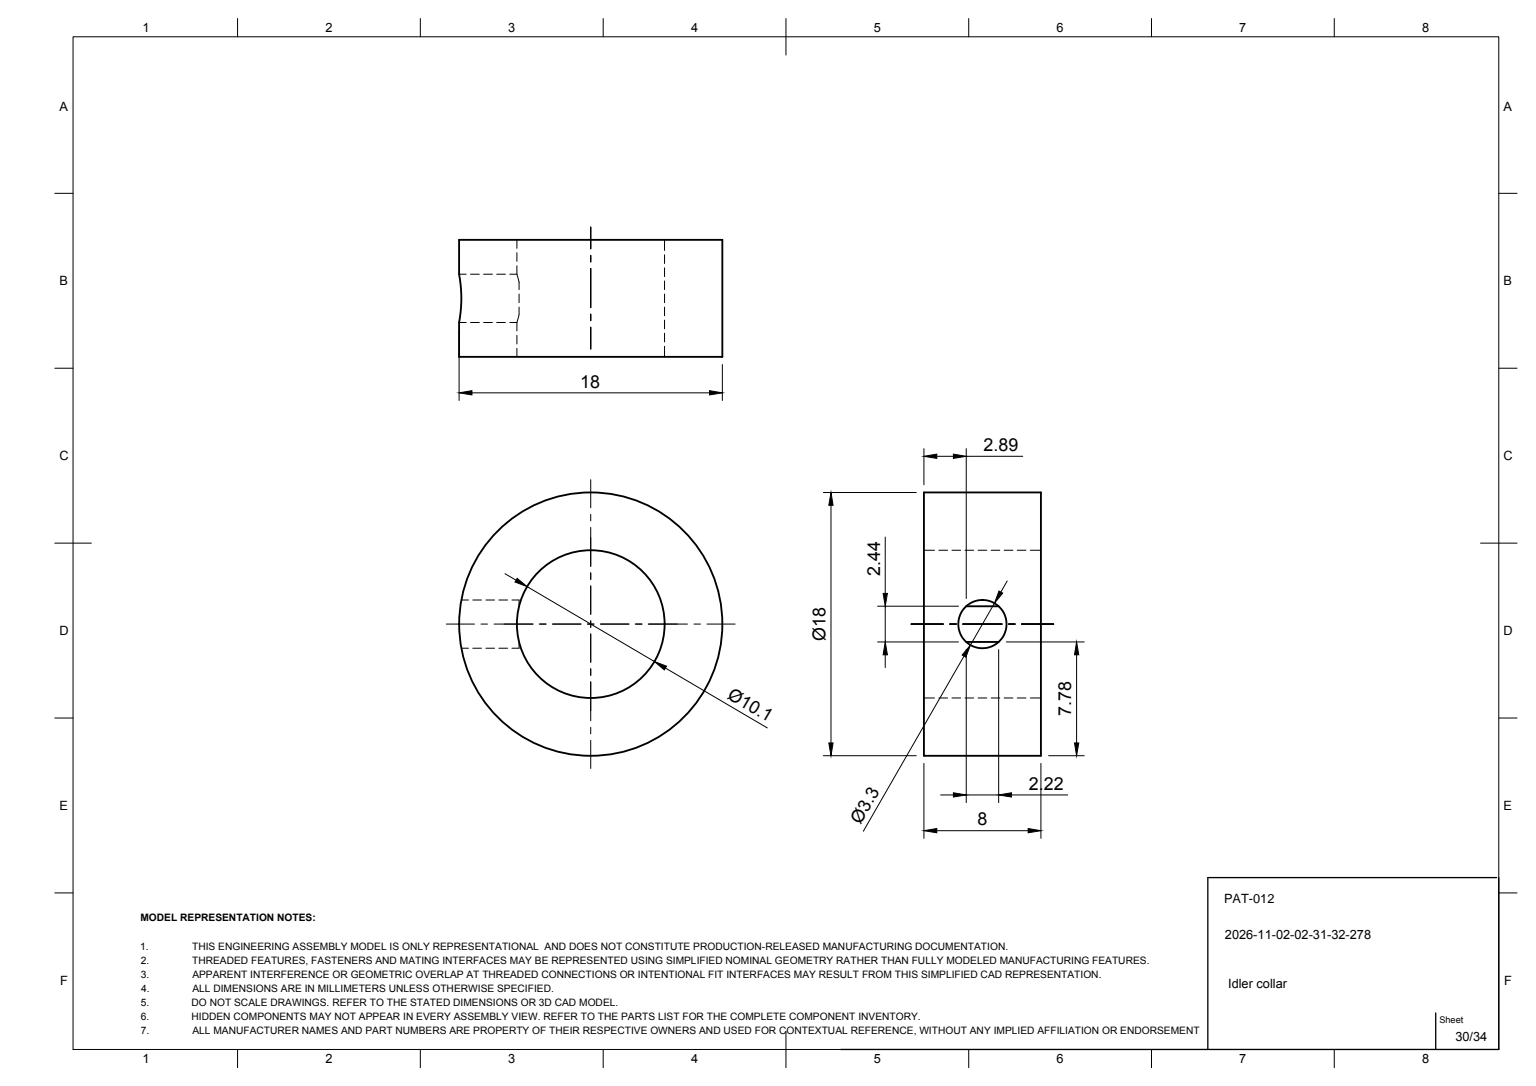
ISO-10303-21;
HEADER;
/* Generated by software containing ST-Developer
 * from STEP Tools, Inc. (www.steptools.com) 
 */

FILE_DESCRIPTION(
/* description */ ('Belt tensioner idler arm'),
/* implementation_level */ '2;1');

FILE_NAME(
/* name */ 'Idler collar.step',
/* time_stamp */ '2026-10-28T03:22:15-07:00',
/* author */ (''),
/* organization */ (''),
/* preprocessor_version */ 'ST-DEVELOPER v20.2',
/* originating_system */ 'Autodesk Translation Framework v15.17.0.0',
/* authorisation */ '');

FILE_SCHEMA (('AUTOMOTIVE_DESIGN { 1 0 10303 214 3 1 1 }'));
ENDSEC;

DATA;
#10=MECHANICAL_DESIGN_GEOMETRIC_PRESENTATION_REPRESENTATION('',(#480),#12779);
#352=B_SPLINE_CURVE_WITH_KNOTS('',3,(#11799,#11800,#11801,#11802,#11803,
#11804,#11805,#11806,#11807,#11808,#11809,#11810,#11811,#11812),
 .UNSPECIFIED.,.F.,.F.,(4,2,2,2,2,2,4),(0.618551524396289,0.626563103102765,
0.689203386094988,0.751843669087211,0.814483952079434,0.877124235071657,
0.885135813778134),.UNSPECIFIED.);
#353=B_SPLINE_CURVE_WITH_KNOTS('',3,(#11816,#11817,#11818,#11819,#11820,
#11821,#11822,#11823),.UNSPECIFIED.,.F.,.F.,(4,2,2,4),(0.250614556362404,
0.313254839354627,0.37589512234685,0.383906701053325),.UNSPECIFIED.);
#354=B_SPLINE_CURVE_WITH_KNOTS('',3,(#11827,#11828,#11829,#11830,#11831,
#11832,#11833,#11834,#11835,#11836,#11837,#11838,#11839,#11840,#11841,#11842,
#11843,#11844,#11845,#11846,#11847,#11848,#11849,#11850,#11851,#11852),
 .UNSPECIFIED.,.F.,.F.,(4,2,2,2,2,2,2,2,2,2,2,2,4),(0.,0.0623062782223143,
0.124612556444629,0.186916384615149,0.249220212785669,0.31152404095619,
0.37382786912671,0.436134147349024,0.498440425571339,0.560746703793653,
0.623052982015967,0.685356810186488,0.747660638357008),.UNSPECIFIED.);
#355=B_SPLINE_CURVE_WITH_KNOTS('',3,(#11853,#11854,#11855,#11856,#11857,
#11858,#11859,#11860,#11861,#11862),.UNSPECIFIED.,.F.,.F.,(4,2,2,2,4),(0.747660638357008,
0.809964466527529,0.872268294698049,0.934574572920363,0.996880851142677),
 .UNSPECIFIED.);
#356=B_SPLINE_CURVE_WITH_KNOTS('',3,(#11863,#11864,#11865,#11866,#11867,
#11868,#11869,#11870),.UNSPECIFIED.,.F.,.F.,(4,2,2,4),(0.117322411671483,
0.125333990377958,0.187974273370181,0.250614556362404),.UNSPECIFIED.);
#404=SHAPE_REPRESENTATION_RELATIONSHIP('SRR','None',#12953,#438);
#438=ADVANCED_BREP_SHAPE_REPRESENTATION('',(#519),#12770);
#480=STYLED_ITEM('',(#13177),#519);
#519=MANIFOLD_SOLID_BREP('Body1',#6217);
#640=FACE_BOUND('',#1583,.T.);
#641=FACE_BOUND('',#1585,.T.);
#642=FACE_BOUND('',#1587,.T.);
#643=FACE_BOUND('',#1589,.T.);
#798=PLANE('',#7168);
#799=PLANE('',#7172);
#800=PLANE('',#7179);
#801=PLANE('',#7180);
#1099=FACE_OUTER_BOUND('',#1579,.T.);
#1100=FACE_OUTER_BOUND('',#1580,.T.);
#1101=FACE_OUTER_BOUND('',#1581,.T.);
#1102=FACE_OUTER_BOUND('',#1582,.T.);
#1103=FACE_OUTER_BOUND('',#1584,.T.);
#1104=FACE_OUTER_BOUND('',#1586,.T.);
#1105=FACE_OUTER_BOUND('',#1588,.T.);
#1579=EDGE_LOOP('',(#5156,#5157));
#1580=EDGE_LOOP('',(#5158,#5159,#5160,#5161,#5162,#5163,#5164,#5165,#5166));
#1581=EDGE_LOOP('',(#5167,#5168));
#1582=EDGE_LOOP('',(#5169,#5170,#5171,#5172));
#1583=EDGE_LOOP('',(#5173,#5174,#5175,#5176,#5177));
#1584=EDGE_LOOP('',(#5178,#5179,#5180,#5181));
#1585=EDGE_LOOP('',(#5182,#5183));
#1586=EDGE_LOOP('',(#5184));
#1587=EDGE_LOOP('',(#5185));
#1588=EDGE_LOOP('',(#5186));
#1589=EDGE_LOOP('',(#5187));
#1950=LINE('',#11795,#2299);
#1951=LINE('',#11825,#2300);
#1952=LINE('',#11872,#2301);
#1953=LINE('',#11877,#2302);
#1954=LINE('',#11883,#2303);
#2299=VECTOR('',#8810,1.);
#2300=VECTOR('',#8817,0.165);
#2301=VECTOR('',#8820,1.);
#2302=VECTOR('',#8825,0.505000000000001);
#2303=VECTOR('',#8832,0.9);
#2649=CIRCLE('',#7169,0.165);
#2650=CIRCLE('',#7171,0.165);
#2651=CIRCLE('',#7174,0.505000000000001);
#2652=CIRCLE('',#7175,0.505000000000001);
#2653=CIRCLE('',#7177,0.9);
#2654=CIRCLE('',#7178,0.9);
#3127=VERTEX_POINT('',#11793);
#3128=VERTEX_POINT('',#11794);
#3129=VERTEX_POINT('',#11798);
#3130=VERTEX_POINT('',#11813);
#3131=VERTEX_POINT('',#11815);
#3132=VERTEX_POINT('',#11824);
#3133=VERTEX_POINT('',#11826);
#3134=VERTEX_POINT('',#11874);
#3135=VERTEX_POINT('',#11876);
#3136=VERTEX_POINT('',#11880);
#3137=VERTEX_POINT('',#11882);
#3833=EDGE_CURVE('',#3127,#3128,#1950,.T.);
#3834=EDGE_CURVE('',#3127,#3128,#2649,.T.);
#3835=EDGE_CURVE('',#3129,#3127,#352,.T.);
#3836=EDGE_CURVE('',#3130,#3129,#2650,.T.);
#3837=EDGE_CURVE('',#3131,#3130,#353,.T.);
#3838=EDGE_CURVE('',#3131,#3132,#1951,.T.);
#3839=EDGE_CURVE('',#3133,#3132,#354,.T.);
#3840=EDGE_CURVE('',#3132,#3133,#355,.T.);
#3841=EDGE_CURVE('',#3128,#3131,#356,.T.);
#3842=EDGE_CURVE('',#3130,#3129,#1952,.T.);
#3843=EDGE_CURVE('',#3134,#3134,#2651,.T.);
#3844=EDGE_CURVE('',#3134,#3135,#1953,.T.);
#3845=EDGE_CURVE('',#3135,#3135,#2652,.T.);
#3846=EDGE_CURVE('',#3136,#3136,#2653,.T.);
#3847=EDGE_CURVE('',#3136,#3137,#1954,.T.);
#3848=EDGE_CURVE('',#3137,#3137,#2654,.T.);
#5156=ORIENTED_EDGE('',*,*,#3833,.F.);
#5157=ORIENTED_EDGE('',*,*,#3834,.T.);
#5158=ORIENTED_EDGE('',*,*,#3835,.F.);
#5159=ORIENTED_EDGE('',*,*,#3836,.F.);
#5160=ORIENTED_EDGE('',*,*,#3837,.F.);
#5161=ORIENTED_EDGE('',*,*,#3838,.T.);
#5162=ORIENTED_EDGE('',*,*,#3839,.F.);
#5163=ORIENTED_EDGE('',*,*,#3840,.F.);
#5164=ORIENTED_EDGE('',*,*,#3838,.F.);
#5165=ORIENTED_EDGE('',*,*,#3841,.F.);
#5166=ORIENTED_EDGE('',*,*,#3834,.F.);
#5167=ORIENTED_EDGE('',*,*,#3842,.F.);
#5168=ORIENTED_EDGE('',*,*,#3836,.T.);
#5169=ORIENTED_EDGE('',*,*,#3843,.F.);
#5170=ORIENTED_EDGE('',*,*,#3844,.T.);
#5171=ORIENTED_EDGE('',*,*,#3845,.T.);
#5172=ORIENTED_EDGE('',*,*,#3844,.F.);
#5173=ORIENTED_EDGE('',*,*,#3841,.T.);
#5174=ORIENTED_EDGE('',*,*,#3837,.T.);
#5175=ORIENTED_EDGE('',*,*,#3842,.T.);
#5176=ORIENTED_EDGE('',*,*,#3835,.T.);
#5177=ORIENTED_EDGE('',*,*,#3833,.T.);
#5178=ORIENTED_EDGE('',*,*,#3846,.F.);
#5179=ORIENTED_EDGE('',*,*,#3847,.T.);
#5180=ORIENTED_EDGE('',*,*,#3848,.T.);
#5181=ORIENTED_EDGE('',*,*,#3847,.F.);
#5182=ORIENTED_EDGE('',*,*,#3839,.T.);
#5183=ORIENTED_EDGE('',*,*,#3840,.T.);
#5184=ORIENTED_EDGE('',*,*,#3846,.T.);
#5185=ORIENTED_EDGE('',*,*,#3843,.T.);
#5186=ORIENTED_EDGE('',*,*,#3848,.F.);
#5187=ORIENTED_EDGE('',*,*,#3845,.F.);
#5752=CYLINDRICAL_SURFACE('',#7170,0.165);
#5753=CYLINDRICAL_SURFACE('',#7173,0.505000000000001);
#5754=CYLINDRICAL_SURFACE('',#7176,0.9);
#6076=ADVANCED_FACE('',(#1099),#798,.T.);
#6077=ADVANCED_FACE('',(#1100),#5752,.F.);
#6078=ADVANCED_FACE('',(#1101),#799,.T.);
#6079=ADVANCED_FACE('',(#1102,#640),#5753,.F.);
#6080=ADVANCED_FACE('',(#1103,#641),#5754,.T.);
#6081=ADVANCED_FACE('',(#1104,#642),#800,.T.);
#6082=ADVANCED_FACE('',(#1105,#643),#801,.F.);
#6217=CLOSED_SHELL('',(#6076,#6077,#6078,#6079,#6080,#6081,#6082));
#7167=AXIS2_PLACEMENT_3D('',#11791,#8806,#8807);
#7168=AXIS2_PLACEMENT_3D('',#11792,#8808,#8809);
#7169=AXIS2_PLACEMENT_3D('',#11796,#8811,#8812);
#7170=AXIS2_PLACEMENT_3D('',#11797,#8813,#8814);
#7171=AXIS2_PLACEMENT_3D('',#11814,#8815,#8816);
#7172=AXIS2_PLACEMENT_3D('',#11871,#8818,#8819);
#7173=AXIS2_PLACEMENT_3D('',#11873,#8821,#8822);
#7174=AXIS2_PLACEMENT_3D('',#11875,#8823,#8824);
#7175=AXIS2_PLACEMENT_3D('',#11878,#8826,#8827);
#7176=AXIS2_PLACEMENT_3D('',#11879,#8828,#8829);
#7177=AXIS2_PLACEMENT_3D('',#11881,#8830,#8831);
#7178=AXIS2_PLACEMENT_3D('',#11884,#8833,#8834);
#7179=AXIS2_PLACEMENT_3D('',#11885,#8835,#8836);
#7180=AXIS2_PLACEMENT_3D('',#11886,#8837,#8838);
#8806=DIRECTION('axis',(0.,0.,1.));
#8807=DIRECTION('refdir',(1.,0.,0.));
#8808=DIRECTION('center_axis',(1.,0.,0.));
#8809=DIRECTION('ref_axis',(0.,0.,-1.));
#8810=DIRECTION('',(0.,0.,1.));
#8811=DIRECTION('center_axis',(1.,0.,0.));
#8812=DIRECTION('ref_axis',(0.,0.,-1.));
#8813=DIRECTION('center_axis',(1.,0.,0.));
#8814=DIRECTION('ref_axis',(0.,0.,-1.));
#8815=DIRECTION('center_axis',(1.,0.,0.));
#8816=DIRECTION('ref_axis',(0.,0.,-1.));
#8817=DIRECTION('',(1.,0.,0.));
#8818=DIRECTION('center_axis',(1.,0.,0.));
#8819=DIRECTION('ref_axis',(0.,0.,-1.));
#8820=DIRECTION('',(0.,0.,-1.));
#8821=DIRECTION('center_axis',(0.,0.,1.));
#8822=DIRECTION('ref_axis',(1.,0.,0.));
#8823=DIRECTION('center_axis',(0.,0.,-1.));
#8824=DIRECTION('ref_axis',(1.,0.,0.));
#8825=DIRECTION('',(0.,0.,-1.));
#8826=DIRECTION('center_axis',(0.,0.,-1.));
#8827=DIRECTION('ref_axis',(1.,0.,0.));
#8828=DIRECTION('center_axis',(0.,0.,1.));
#8829=DIRECTION('ref_axis',(1.,0.,0.));
#8830=DIRECTION('center_axis',(0.,0.,1.));
#8831=DIRECTION('ref_axis',(1.,0.,0.));
#8832=DIRECTION('',(0.,0.,-1.));
#8833=DIRECTION('center_axis',(0.,0.,1.));
#8834=DIRECTION('ref_axis',(1.,0.,0.));
#8835=DIRECTION('center_axis',(0.,0.,1.));
#8836=DIRECTION('ref_axis',(1.,0.,0.));
#8837=DIRECTION('center_axis',(0.,0.,1.));
#8838=DIRECTION('ref_axis',(1.,0.,0.));
#11791=CARTESIAN_POINT('',(0.,0.,0.));
#11792=CARTESIAN_POINT('Origin',(9.49,0.,4.65));
#11793=CARTESIAN_POINT('',(9.49,0.122167917228709,4.53909463493591));
#11794=CARTESIAN_POINT('',(9.49,0.122167917228709,4.76090536506409));
#11795=CARTESIAN_POINT('',(9.49,0.122167917228709,4.25));
#11796=CARTESIAN_POINT('Origin',(9.49,0.,4.65));
#11797=CARTESIAN_POINT('Origin',(9.49,0.,4.65));
#11798=CARTESIAN_POINT('',(9.49,-0.122167917228709,4.53909463493591));
#11799=CARTESIAN_POINT('Ctrl Pts',(9.49,-0.122167917228708,4.53909463493591));
#11800=CARTESIAN_POINT('Ctrl Pts',(9.49044853167999,-0.120368913626297,
4.53711294069536));
#11801=CARTESIAN_POINT('Ctrl Pts',(9.49089524537169,-0.118534896565231,
4.53518965877367));
#11802=CARTESIAN_POINT('Ctrl Pts',(9.49479501553165,-0.102111993019358,
4.5187667552278));
#11803=CARTESIAN_POINT('Ctrl Pts',(9.49844251460759,-0.0836597150224316,
4.50609154388858));
#11804=CARTESIAN_POINT('Ctrl Pts',(9.50357781976106,-0.0430495960471595,
4.48920409039234));
#11805=CARTESIAN_POINT('Ctrl Pts',(9.505,-0.020880094330741,4.485));
#11806=CARTESIAN_POINT('Ctrl Pts',(9.505,0.020880094330741,4.485));
#11807=CARTESIAN_POINT('Ctrl Pts',(9.50357781976106,0.0430495960471595,
4.48920409039234));
#11808=CARTESIAN_POINT('Ctrl Pts',(9.49844251460759,0.0836597150224316,
4.50609154388858));
#11809=CARTESIAN_POINT('Ctrl Pts',(9.49479501553165,0.102111993019358,4.5187667552278));
#11810=CARTESIAN_POINT('Ctrl Pts',(9.49089524537169,0.118534896565231,4.53518965877367));
#11811=CARTESIAN_POINT('Ctrl Pts',(9.49044853167999,0.120368913626297,4.53711294069536));
#11812=CARTESIAN_POINT('Ctrl Pts',(9.49,0.122167917228708,4.53909463493591));
#11813=CARTESIAN_POINT('',(9.49,-0.122167917228709,4.76090536506409));
#11814=CARTESIAN_POINT('Origin',(9.49,0.,4.65));
#11815=CARTESIAN_POINT('',(9.505,-1.70422299968729E-17,4.815));
#11816=CARTESIAN_POINT('Ctrl Pts',(9.505,-2.77555756156289E-17,4.815));
#11817=CARTESIAN_POINT('Ctrl Pts',(9.505,-0.020880094330741,4.815));
#11818=CARTESIAN_POINT('Ctrl Pts',(9.50357781976106,-0.0430495960471595,
4.81079590960766));
#11819=CARTESIAN_POINT('Ctrl Pts',(9.49844251460759,-0.0836597150224317,
4.79390845611142));
#11820=CARTESIAN_POINT('Ctrl Pts',(9.49479501553165,-0.102111993019358,
4.7812332447722));
#11821=CARTESIAN_POINT('Ctrl Pts',(9.49089524537169,-0.118534896565231,
4.76481034122633));
#11822=CARTESIAN_POINT('Ctrl Pts',(9.49044853167999,-0.120368913626296,
4.76288705930464));
#11823=CARTESIAN_POINT('Ctrl Pts',(9.49,-0.122167917228708,4.76090536506409));
#11824=CARTESIAN_POINT('',(9.9,-2.02066721859313E-17,4.815));
#11825=CARTESIAN_POINT('',(9.49,-2.02066721859313E-17,4.815));
#11826=CARTESIAN_POINT('',(9.88474572618352,0.165,4.65));
#11827=CARTESIAN_POINT('Ctrl Pts',(9.88474572618352,0.165,4.65));
#11828=CARTESIAN_POINT('Ctrl Pts',(9.88474572618352,0.165,4.62923124059256));
#11829=CARTESIAN_POINT('Ctrl Pts',(9.88555275950526,0.160839719007584,4.60711110492666));
#11830=CARTESIAN_POINT('Ctrl Pts',(9.88844864815004,0.14398647021669,4.56647293736623));
#11831=CARTESIAN_POINT('Ctrl Pts',(9.89049360485164,0.131295993814186,4.54795075602263));
#11832=CARTESIAN_POINT('Ctrl Pts',(9.89431723432394,0.102049819008125,4.51870458121656));
#11833=CARTESIAN_POINT('Ctrl Pts',(9.89634708889954,0.0835273920906821,
4.50601365401642));
#11834=CARTESIAN_POINT('Ctrl Pts',(9.89920827186059,0.0428883760934128,
4.48916007816136));
#11835=CARTESIAN_POINT('Ctrl Pts',(9.9,0.0207679427235068,4.485));
#11836=CARTESIAN_POINT('Ctrl Pts',(9.9,-0.0207679427235068,4.485));
#11837=CARTESIAN_POINT('Ctrl Pts',(9.89920827186059,-0.0428883760934128,
4.48916007816136));
#11838=CARTESIAN_POINT('Ctrl Pts',(9.89634708889954,-0.0835273920906821,
4.50601365401642));
#11839=CARTESIAN_POINT('Ctrl Pts',(9.89431723432394,-0.102049819008125,
4.51870458121656));
#11840=CARTESIAN_POINT('Ctrl Pts',(9.89049360485164,-0.131295993814186,
4.54795075602263));
#11841=CARTESIAN_POINT('Ctrl Pts',(9.88844864815004,-0.14398647021669,4.56647293736623));
#11842=CARTESIAN_POINT('Ctrl Pts',(9.88555275950526,-0.160839719007584,
4.60711110492666));
#11843=CARTESIAN_POINT('Ctrl Pts',(9.88474572618352,-0.165,4.62923124059256));
#11844=CARTESIAN_POINT('Ctrl Pts',(9.88474572618352,-0.165,4.67076875940744));
#11845=CARTESIAN_POINT('Ctrl Pts',(9.88555275950526,-0.160839719007584,
4.69288889507335));
#11846=CARTESIAN_POINT('Ctrl Pts',(9.88844864815004,-0.14398647021669,4.73352706263377));
#11847=CARTESIAN_POINT('Ctrl Pts',(9.89049360485164,-0.131295993814186,
4.75204924397737));
#11848=CARTESIAN_POINT('Ctrl Pts',(9.89431723432394,-0.102049819008125,
4.78129541878344));
#11849=CARTESIAN_POINT('Ctrl Pts',(9.89634708889954,-0.0835273920906821,
4.79398634598358));
#11850=CARTESIAN_POINT('Ctrl Pts',(9.89920827186059,-0.0428883760934128,
4.81083992183864));
#11851=CARTESIAN_POINT('Ctrl Pts',(9.9,-0.0207679427235068,4.815));
#11852=CARTESIAN_POINT('Ctrl Pts',(9.9,0.,4.815));
#11853=CARTESIAN_POINT('Ctrl Pts',(9.9,-2.08166817117217E-17,4.815));
#11854=CARTESIAN_POINT('Ctrl Pts',(9.9,0.0207679427235068,4.815));
#11855=CARTESIAN_POINT('Ctrl Pts',(9.89920827186059,0.0428883760934128,
4.81083992183864));
#11856=CARTESIAN_POINT('Ctrl Pts',(9.89634708889954,0.0835273920906821,
4.79398634598358));
#11857=CARTESIAN_POINT('Ctrl Pts',(9.89431723432394,0.102049819008125,4.78129541878344));
#11858=CARTESIAN_POINT('Ctrl Pts',(9.89049360485164,0.131295993814186,4.75204924397737));
#11859=CARTESIAN_POINT('Ctrl Pts',(9.88844864815004,0.14398647021669,4.73352706263377));
#11860=CARTESIAN_POINT('Ctrl Pts',(9.88555275950526,0.160839719007584,4.69288889507335));
#11861=CARTESIAN_POINT('Ctrl Pts',(9.88474572618352,0.165,4.67076875940744));
#11862=CARTESIAN_POINT('Ctrl Pts',(9.88474572618352,0.165,4.65));
#11863=CARTESIAN_POINT('Ctrl Pts',(9.49,0.122167917228708,4.76090536506409));
#11864=CARTESIAN_POINT('Ctrl Pts',(9.49044853167999,0.120368913626296,4.76288705930464));
#11865=CARTESIAN_POINT('Ctrl Pts',(9.49089524537169,0.118534896565231,4.76481034122633));
#11866=CARTESIAN_POINT('Ctrl Pts',(9.49479501553165,0.102111993019358,4.7812332447722));
#11867=CARTESIAN_POINT('Ctrl Pts',(9.49844251460759,0.0836597150224316,
4.79390845611142));
#11868=CARTESIAN_POINT('Ctrl Pts',(9.50357781976106,0.0430495960471595,
4.81079590960766));
#11869=CARTESIAN_POINT('Ctrl Pts',(9.505,0.020880094330741,4.815));
#11870=CARTESIAN_POINT('Ctrl Pts',(9.505,-2.77555756156289E-17,4.815));
#11871=CARTESIAN_POINT('Origin',(9.49,0.,4.65));
#11872=CARTESIAN_POINT('',(9.49,-0.122167917228709,4.25));
#11873=CARTESIAN_POINT('Origin',(9.,0.,4.25));
#11874=CARTESIAN_POINT('',(8.495,-6.18446633569414E-17,5.05));
#11875=CARTESIAN_POINT('Origin',(9.,0.,5.05));
#11876=CARTESIAN_POINT('',(8.495,-6.18446633569414E-17,4.25));
#11877=CARTESIAN_POINT('',(8.495,-6.18446633569414E-17,4.25));
#11878=CARTESIAN_POINT('Origin',(9.,0.,4.25));
#11879=CARTESIAN_POINT('Origin',(9.,0.,4.25));
#11880=CARTESIAN_POINT('',(8.1,-1.10218211923262E-16,5.05));
#11881=CARTESIAN_POINT('Origin',(9.,0.,5.05));
#11882=CARTESIAN_POINT('',(8.1,-1.10218211923262E-16,4.25));
#11883=CARTESIAN_POINT('',(8.1,-1.10218211923262E-16,4.25));
#11884=CARTESIAN_POINT('Origin',(9.,0.,4.25));
#11885=CARTESIAN_POINT('Origin',(9.,0.,5.05));
#11886=CARTESIAN_POINT('Origin',(9.,0.,4.25));
#12730=UNCERTAINTY_MEASURE_WITH_UNIT(LENGTH_MEASURE(0.001),#12780,
'DISTANCE_ACCURACY_VALUE',
'Maximum model space distance between geometric entities at asserted c
onnectivities');
#12739=UNCERTAINTY_MEASURE_WITH_UNIT(LENGTH_MEASURE(0.001),#12780,
'DISTANCE_ACCURACY_VALUE',
'Maximum model space distance between geometric entities at asserted c
onnectivities');
#12770=(
GEOMETRIC_REPRESENTATION_CONTEXT(3)
GLOBAL_UNCERTAINTY_ASSIGNED_CONTEXT((#12730))
GLOBAL_UNIT_ASSIGNED_CONTEXT((#12780,#12782,#12783))
REPRESENTATION_CONTEXT('','3D')
);
#12779=(
GEOMETRIC_REPRESENTATION_CONTEXT(3)
GLOBAL_UNCERTAINTY_ASSIGNED_CONTEXT((#12739))
GLOBAL_UNIT_ASSIGNED_CONTEXT((#12780,#12782,#12783))
REPRESENTATION_CONTEXT('','3D')
);
#12780=(
LENGTH_UNIT()
NAMED_UNIT(*)
SI_UNIT(.CENTI.,.METRE.)
);
#12782=(
NAMED_UNIT(*)
PLANE_ANGLE_UNIT()
SI_UNIT($,.RADIAN.)
);
#12783=(
NAMED_UNIT(*)
SI_UNIT($,.STERADIAN.)
SOLID_ANGLE_UNIT()
);
#12814=SHAPE_DEFINITION_REPRESENTATION(#12882,#12953);
#12882=PRODUCT_DEFINITION_SHAPE('',$,#12993);
#12953=SHAPE_REPRESENTATION('',(#7167),#12770);
#12962=PRODUCT_DEFINITION_CONTEXT('part definition',#13081,'design');
#12993=PRODUCT_DEFINITION('Idler collar','Idler collar',#13032,#12962);
#13032=PRODUCT_DEFINITION_FORMATION('',$,#13113);
#13081=APPLICATION_CONTEXT(
'Core Data for Automotive Mechanical Design Process');
#13082=PRODUCT_CONTEXT('part definition',#13081,'mechanical');
#13113=PRODUCT('Idler collar','Idler collar','Idler collar',(#13082));
#13171=COLOUR_RGB('Sky Blue',0.24,0.69,0.87);
#13172=FILL_AREA_STYLE_COLOUR('',#13171);
#13173=FILL_AREA_STYLE('',(#13172));
#13174=SURFACE_STYLE_FILL_AREA(#13173);
#13175=SURFACE_SIDE_STYLE('',(#13174));
#13176=SURFACE_STYLE_USAGE(.BOTH.,#13175);
#13177=PRESENTATION_STYLE_ASSIGNMENT((#13176));
ENDSEC;
END-ISO-10303-21;
